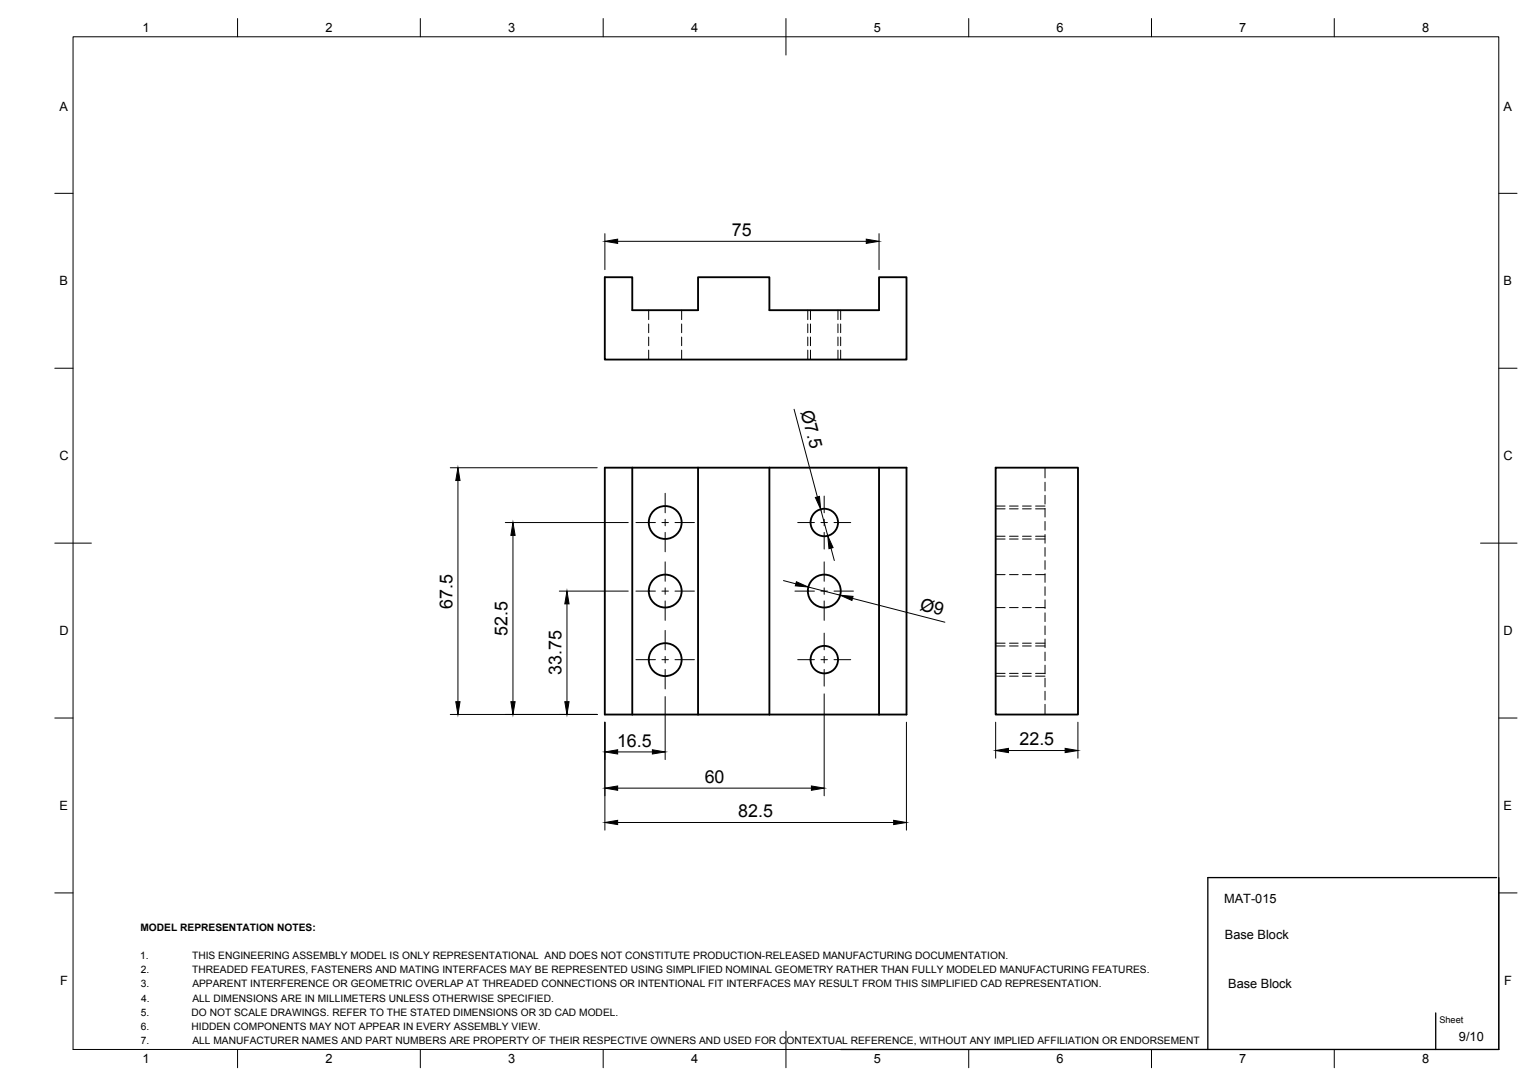
ISO-10303-21;
HEADER;
/* Generated by software containing ST-Developer
 * from STEP Tools, Inc. (www.steptools.com) 
 */

FILE_DESCRIPTION(
/* description */ ('STEP AP214'),
/* implementation_level */ '2;1');

FILE_NAME(
/* name */ 'Base Block.step',
/* time_stamp */ '2026-11-14T06:03:18-08:00',
/* author */ (''),
/* organization */ (''),
/* preprocessor_version */ 'ST-DEVELOPER v20.2',
/* originating_system */ 'Autodesk Translation Framework v15.17.0.0',
/* authorisation */ '');

FILE_SCHEMA (('AUTOMOTIVE_DESIGN { 1 0 10303 214 3 1 1 }'));
ENDSEC;

DATA;
#10=MECHANICAL_DESIGN_GEOMETRIC_PRESENTATION_REPRESENTATION('',(#77),#3206);
#61=SHAPE_REPRESENTATION_RELATIONSHIP('SRR','None',#3244,#69);
#69=ADVANCED_BREP_SHAPE_REPRESENTATION('',(#85),#3203);
#77=STYLED_ITEM('',(#3289),#85);
#85=MANIFOLD_SOLID_BREP('Body1',#1784);
#117=PLANE('',#2002);
#118=PLANE('',#2003);
#119=PLANE('',#2004);
#120=PLANE('',#2005);
#121=PLANE('',#2006);
#122=PLANE('',#2007);
#123=PLANE('',#2008);
#124=PLANE('',#2009);
#125=PLANE('',#2010);
#126=PLANE('',#2011);
#127=PLANE('',#2012);
#128=PLANE('',#2013);
#129=PLANE('',#2014);
#130=PLANE('',#2015);
#168=FACE_BOUND('',#693,.T.);
#169=FACE_BOUND('',#694,.T.);
#170=FACE_BOUND('',#695,.T.);
#171=FACE_BOUND('',#697,.T.);
#172=FACE_BOUND('',#698,.T.);
#173=FACE_BOUND('',#699,.T.);
#174=FACE_BOUND('',#701,.T.);
#175=FACE_BOUND('',#702,.T.);
#176=FACE_BOUND('',#703,.T.);
#177=FACE_BOUND('',#704,.T.);
#178=FACE_BOUND('',#705,.T.);
#179=FACE_BOUND('',#706,.T.);
#244=LINE('',#2930,#389);
#245=LINE('',#2936,#390);
#246=LINE('',#2942,#391);
#247=LINE('',#2948,#392);
#248=LINE('',#2954,#393);
#249=LINE('',#2960,#394);
#250=LINE('',#2965,#395);
#251=LINE('',#2967,#396);
#252=LINE('',#2969,#397);
#253=LINE('',#2970,#398);
#254=LINE('',#2974,#399);
#255=LINE('',#2976,#400);
#256=LINE('',#2978,#401);
#257=LINE('',#2979,#402);
#258=LINE('',#2983,#403);
#259=LINE('',#2985,#404);
#260=LINE('',#2987,#405);
#261=LINE('',#2988,#406);
#262=LINE('',#2991,#407);
#263=LINE('',#2993,#408);
#264=LINE('',#2994,#409);
#265=LINE('',#2997,#410);
#266=LINE('',#2999,#411);
#267=LINE('',#3000,#412);
#268=LINE('',#3002,#413);
#269=LINE('',#3004,#414);
#270=LINE('',#3005,#415);
#271=LINE('',#3007,#416);
#272=LINE('',#3008,#417);
#273=LINE('',#3011,#418);
#274=LINE('',#3012,#419);
#275=LINE('',#3015,#420);
#276=LINE('',#3016,#421);
#277=LINE('',#3018,#422);
#278=LINE('',#3020,#423);
#279=LINE('',#3021,#424);
#280=LINE('',#3023,#425);
#281=LINE('',#3024,#426);
#282=LINE('',#3026,#427);
#283=LINE('',#3028,#428);
#284=LINE('',#3031,#429);
#285=LINE('',#3034,#430);
#389=VECTOR('',#2351,4.5);
#390=VECTOR('',#2358,4.5);
#391=VECTOR('',#2365,4.5);
#392=VECTOR('',#2372,4.5);
#393=VECTOR('',#2379,3.75);
#394=VECTOR('',#2386,3.75);
#395=VECTOR('',#2391,1000.);
#396=VECTOR('',#2392,1000.);
#397=VECTOR('',#2393,1000.);
#398=VECTOR('',#2394,1000.);
#399=VECTOR('',#2397,1000.);
#400=VECTOR('',#2398,1000.);
#401=VECTOR('',#2399,1000.);
#402=VECTOR('',#2400,1000.);
#403=VECTOR('',#2403,1000.);
#404=VECTOR('',#2404,1000.);
#405=VECTOR('',#2405,1000.);
#406=VECTOR('',#2406,1000.);
#407=VECTOR('',#2409,1000.);
#408=VECTOR('',#2410,1000.);
#409=VECTOR('',#2411,1000.);
#410=VECTOR('',#2414,1000.);
#411=VECTOR('',#2415,1000.);
#412=VECTOR('',#2416,1000.);
#413=VECTOR('',#2417,1000.);
#414=VECTOR('',#2418,1000.);
#415=VECTOR('',#2419,1000.);
#416=VECTOR('',#2420,1000.);
#417=VECTOR('',#2421,1000.);
#418=VECTOR('',#2424,1000.);
#419=VECTOR('',#2425,1000.);
#420=VECTOR('',#2428,1000.);
#421=VECTOR('',#2429,1000.);
#422=VECTOR('',#2430,1000.);
#423=VECTOR('',#2431,1000.);
#424=VECTOR('',#2432,1000.);
#425=VECTOR('',#2433,1000.);
#426=VECTOR('',#2434,1000.);
#427=VECTOR('',#2437,1000.);
#428=VECTOR('',#2440,1000.);
#429=VECTOR('',#2445,1000.);
#430=VECTOR('',#2450,1000.);
#497=CYLINDRICAL_SURFACE('',#1984,4.5);
#498=CYLINDRICAL_SURFACE('',#1987,4.5);
#499=CYLINDRICAL_SURFACE('',#1990,4.5);
#500=CYLINDRICAL_SURFACE('',#1993,4.5);
#501=CYLINDRICAL_SURFACE('',#1996,3.75);
#502=CYLINDRICAL_SURFACE('',#1999,3.75);
#565=FACE_OUTER_BOUND('',#686,.T.);
#566=FACE_OUTER_BOUND('',#687,.T.);
#567=FACE_OUTER_BOUND('',#688,.T.);
#568=FACE_OUTER_BOUND('',#689,.T.);
#569=FACE_OUTER_BOUND('',#690,.T.);
#570=FACE_OUTER_BOUND('',#691,.T.);
#571=FACE_OUTER_BOUND('',#692,.T.);
#572=FACE_OUTER_BOUND('',#696,.T.);
#573=FACE_OUTER_BOUND('',#700,.T.);
#574=FACE_OUTER_BOUND('',#707,.T.);
#575=FACE_OUTER_BOUND('',#708,.T.);
#576=FACE_OUTER_BOUND('',#709,.T.);
#577=FACE_OUTER_BOUND('',#710,.T.);
#578=FACE_OUTER_BOUND('',#711,.T.);
#579=FACE_OUTER_BOUND('',#712,.T.);
#580=FACE_OUTER_BOUND('',#713,.T.);
#581=FACE_OUTER_BOUND('',#714,.T.);
#582=FACE_OUTER_BOUND('',#715,.T.);
#583=FACE_OUTER_BOUND('',#716,.T.);
#584=FACE_OUTER_BOUND('',#717,.T.);
#686=EDGE_LOOP('',(#1433,#1434,#1435,#1436));
#687=EDGE_LOOP('',(#1437,#1438,#1439,#1440));
#688=EDGE_LOOP('',(#1441,#1442,#1443,#1444));
#689=EDGE_LOOP('',(#1445,#1446,#1447,#1448));
#690=EDGE_LOOP('',(#1449,#1450,#1451,#1452));
#691=EDGE_LOOP('',(#1453,#1454,#1455,#1456));
#692=EDGE_LOOP('',(#1457,#1458,#1459,#1460));
#693=EDGE_LOOP('',(#1461));
#694=EDGE_LOOP('',(#1462));
#695=EDGE_LOOP('',(#1463));
#696=EDGE_LOOP('',(#1464,#1465,#1466,#1467));
#697=EDGE_LOOP('',(#1468));
#698=EDGE_LOOP('',(#1469));
#699=EDGE_LOOP('',(#1470));
#700=EDGE_LOOP('',(#1471,#1472,#1473,#1474));
#701=EDGE_LOOP('',(#1475));
#702=EDGE_LOOP('',(#1476));
#703=EDGE_LOOP('',(#1477));
#704=EDGE_LOOP('',(#1478));
#705=EDGE_LOOP('',(#1479));
#706=EDGE_LOOP('',(#1480));
#707=EDGE_LOOP('',(#1481,#1482,#1483,#1484));
#708=EDGE_LOOP('',(#1485,#1486,#1487,#1488,#1489,#1490,#1491,#1492,#1493,
#1494,#1495,#1496));
#709=EDGE_LOOP('',(#1497,#1498,#1499,#1500));
#710=EDGE_LOOP('',(#1501,#1502,#1503,#1504,#1505,#1506,#1507,#1508,#1509,
#1510,#1511,#1512));
#711=EDGE_LOOP('',(#1513,#1514,#1515,#1516));
#712=EDGE_LOOP('',(#1517,#1518,#1519,#1520));
#713=EDGE_LOOP('',(#1521,#1522,#1523,#1524));
#714=EDGE_LOOP('',(#1525,#1526,#1527,#1528));
#715=EDGE_LOOP('',(#1529,#1530,#1531,#1532));
#716=EDGE_LOOP('',(#1533,#1534,#1535,#1536));
#717=EDGE_LOOP('',(#1537,#1538,#1539,#1540));
#801=CIRCLE('',#1985,4.5);
#802=CIRCLE('',#1986,4.5);
#803=CIRCLE('',#1988,4.5);
#804=CIRCLE('',#1989,4.5);
#805=CIRCLE('',#1991,4.5);
#806=CIRCLE('',#1992,4.5);
#807=CIRCLE('',#1994,4.5);
#808=CIRCLE('',#1995,4.5);
#809=CIRCLE('',#1997,3.75);
#810=CIRCLE('',#1998,3.75);
#811=CIRCLE('',#2000,3.75);
#812=CIRCLE('',#2001,3.75);
#906=VERTEX_POINT('',#2927);
#907=VERTEX_POINT('',#2929);
#908=VERTEX_POINT('',#2933);
#909=VERTEX_POINT('',#2935);
#910=VERTEX_POINT('',#2939);
#911=VERTEX_POINT('',#2941);
#912=VERTEX_POINT('',#2945);
#913=VERTEX_POINT('',#2947);
#914=VERTEX_POINT('',#2951);
#915=VERTEX_POINT('',#2953);
#916=VERTEX_POINT('',#2957);
#917=VERTEX_POINT('',#2959);
#918=VERTEX_POINT('',#2963);
#919=VERTEX_POINT('',#2964);
#920=VERTEX_POINT('',#2966);
#921=VERTEX_POINT('',#2968);
#922=VERTEX_POINT('',#2972);
#923=VERTEX_POINT('',#2973);
#924=VERTEX_POINT('',#2975);
#925=VERTEX_POINT('',#2977);
#926=VERTEX_POINT('',#2981);
#927=VERTEX_POINT('',#2982);
#928=VERTEX_POINT('',#2984);
#929=VERTEX_POINT('',#2986);
#930=VERTEX_POINT('',#2990);
#931=VERTEX_POINT('',#2992);
#932=VERTEX_POINT('',#2996);
#933=VERTEX_POINT('',#2998);
#934=VERTEX_POINT('',#3001);
#935=VERTEX_POINT('',#3003);
#936=VERTEX_POINT('',#3006);
#937=VERTEX_POINT('',#3010);
#938=VERTEX_POINT('',#3014);
#939=VERTEX_POINT('',#3017);
#940=VERTEX_POINT('',#3019);
#941=VERTEX_POINT('',#3022);
#1095=EDGE_CURVE('',#906,#906,#801,.T.);
#1096=EDGE_CURVE('',#906,#907,#244,.T.);
#1097=EDGE_CURVE('',#907,#907,#802,.T.);
#1098=EDGE_CURVE('',#908,#908,#803,.T.);
#1099=EDGE_CURVE('',#908,#909,#245,.T.);
#1100=EDGE_CURVE('',#909,#909,#804,.T.);
#1101=EDGE_CURVE('',#910,#910,#805,.T.);
#1102=EDGE_CURVE('',#910,#911,#246,.T.);
#1103=EDGE_CURVE('',#911,#911,#806,.T.);
#1104=EDGE_CURVE('',#912,#912,#807,.T.);
#1105=EDGE_CURVE('',#912,#913,#247,.T.);
#1106=EDGE_CURVE('',#913,#913,#808,.T.);
#1107=EDGE_CURVE('',#914,#914,#809,.T.);
#1108=EDGE_CURVE('',#914,#915,#248,.T.);
#1109=EDGE_CURVE('',#915,#915,#810,.T.);
#1110=EDGE_CURVE('',#916,#916,#811,.T.);
#1111=EDGE_CURVE('',#916,#917,#249,.T.);
#1112=EDGE_CURVE('',#917,#917,#812,.T.);
#1113=EDGE_CURVE('',#918,#919,#250,.T.);
#1114=EDGE_CURVE('',#919,#920,#251,.T.);
#1115=EDGE_CURVE('',#920,#921,#252,.T.);
#1116=EDGE_CURVE('',#921,#918,#253,.T.);
#1117=EDGE_CURVE('',#922,#923,#254,.T.);
#1118=EDGE_CURVE('',#923,#924,#255,.T.);
#1119=EDGE_CURVE('',#924,#925,#256,.T.);
#1120=EDGE_CURVE('',#925,#922,#257,.T.);
#1121=EDGE_CURVE('',#926,#927,#258,.T.);
#1122=EDGE_CURVE('',#928,#926,#259,.T.);
#1123=EDGE_CURVE('',#929,#928,#260,.T.);
#1124=EDGE_CURVE('',#927,#929,#261,.T.);
#1125=EDGE_CURVE('',#930,#927,#262,.T.);
#1126=EDGE_CURVE('',#931,#930,#263,.T.);
#1127=EDGE_CURVE('',#931,#926,#264,.T.);
#1128=EDGE_CURVE('',#932,#929,#265,.T.);
#1129=EDGE_CURVE('',#933,#932,#266,.T.);
#1130=EDGE_CURVE('',#933,#918,#267,.T.);
#1131=EDGE_CURVE('',#934,#921,#268,.T.);
#1132=EDGE_CURVE('',#935,#934,#269,.T.);
#1133=EDGE_CURVE('',#935,#924,#270,.T.);
#1134=EDGE_CURVE('',#936,#923,#271,.T.);
#1135=EDGE_CURVE('',#930,#936,#272,.T.);
#1136=EDGE_CURVE('',#937,#928,#273,.T.);
#1137=EDGE_CURVE('',#932,#937,#274,.T.);
#1138=EDGE_CURVE('',#938,#931,#275,.T.);
#1139=EDGE_CURVE('',#938,#922,#276,.T.);
#1140=EDGE_CURVE('',#939,#925,#277,.T.);
#1141=EDGE_CURVE('',#940,#939,#278,.T.);
#1142=EDGE_CURVE('',#940,#920,#279,.T.);
#1143=EDGE_CURVE('',#941,#919,#280,.T.);
#1144=EDGE_CURVE('',#937,#941,#281,.T.);
#1145=EDGE_CURVE('',#940,#934,#282,.T.);
#1146=EDGE_CURVE('',#935,#939,#283,.T.);
#1147=EDGE_CURVE('',#933,#941,#284,.T.);
#1148=EDGE_CURVE('',#938,#936,#285,.T.);
#1433=ORIENTED_EDGE('',*,*,#1095,.T.);
#1434=ORIENTED_EDGE('',*,*,#1096,.T.);
#1435=ORIENTED_EDGE('',*,*,#1097,.F.);
#1436=ORIENTED_EDGE('',*,*,#1096,.F.);
#1437=ORIENTED_EDGE('',*,*,#1098,.T.);
#1438=ORIENTED_EDGE('',*,*,#1099,.T.);
#1439=ORIENTED_EDGE('',*,*,#1100,.F.);
#1440=ORIENTED_EDGE('',*,*,#1099,.F.);
#1441=ORIENTED_EDGE('',*,*,#1101,.T.);
#1442=ORIENTED_EDGE('',*,*,#1102,.T.);
#1443=ORIENTED_EDGE('',*,*,#1103,.F.);
#1444=ORIENTED_EDGE('',*,*,#1102,.F.);
#1445=ORIENTED_EDGE('',*,*,#1104,.T.);
#1446=ORIENTED_EDGE('',*,*,#1105,.T.);
#1447=ORIENTED_EDGE('',*,*,#1106,.F.);
#1448=ORIENTED_EDGE('',*,*,#1105,.F.);
#1449=ORIENTED_EDGE('',*,*,#1107,.T.);
#1450=ORIENTED_EDGE('',*,*,#1108,.T.);
#1451=ORIENTED_EDGE('',*,*,#1109,.F.);
#1452=ORIENTED_EDGE('',*,*,#1108,.F.);
#1453=ORIENTED_EDGE('',*,*,#1110,.T.);
#1454=ORIENTED_EDGE('',*,*,#1111,.T.);
#1455=ORIENTED_EDGE('',*,*,#1112,.F.);
#1456=ORIENTED_EDGE('',*,*,#1111,.F.);
#1457=ORIENTED_EDGE('',*,*,#1113,.T.);
#1458=ORIENTED_EDGE('',*,*,#1114,.T.);
#1459=ORIENTED_EDGE('',*,*,#1115,.T.);
#1460=ORIENTED_EDGE('',*,*,#1116,.T.);
#1461=ORIENTED_EDGE('',*,*,#1107,.F.);
#1462=ORIENTED_EDGE('',*,*,#1110,.F.);
#1463=ORIENTED_EDGE('',*,*,#1104,.F.);
#1464=ORIENTED_EDGE('',*,*,#1117,.T.);
#1465=ORIENTED_EDGE('',*,*,#1118,.T.);
#1466=ORIENTED_EDGE('',*,*,#1119,.T.);
#1467=ORIENTED_EDGE('',*,*,#1120,.T.);
#1468=ORIENTED_EDGE('',*,*,#1095,.F.);
#1469=ORIENTED_EDGE('',*,*,#1101,.F.);
#1470=ORIENTED_EDGE('',*,*,#1098,.F.);
#1471=ORIENTED_EDGE('',*,*,#1121,.F.);
#1472=ORIENTED_EDGE('',*,*,#1122,.F.);
#1473=ORIENTED_EDGE('',*,*,#1123,.F.);
#1474=ORIENTED_EDGE('',*,*,#1124,.F.);
#1475=ORIENTED_EDGE('',*,*,#1109,.T.);
#1476=ORIENTED_EDGE('',*,*,#1103,.T.);
#1477=ORIENTED_EDGE('',*,*,#1097,.T.);
#1478=ORIENTED_EDGE('',*,*,#1100,.T.);
#1479=ORIENTED_EDGE('',*,*,#1106,.T.);
#1480=ORIENTED_EDGE('',*,*,#1112,.T.);
#1481=ORIENTED_EDGE('',*,*,#1121,.T.);
#1482=ORIENTED_EDGE('',*,*,#1125,.F.);
#1483=ORIENTED_EDGE('',*,*,#1126,.F.);
#1484=ORIENTED_EDGE('',*,*,#1127,.T.);
#1485=ORIENTED_EDGE('',*,*,#1124,.T.);
#1486=ORIENTED_EDGE('',*,*,#1128,.F.);
#1487=ORIENTED_EDGE('',*,*,#1129,.F.);
#1488=ORIENTED_EDGE('',*,*,#1130,.T.);
#1489=ORIENTED_EDGE('',*,*,#1116,.F.);
#1490=ORIENTED_EDGE('',*,*,#1131,.F.);
#1491=ORIENTED_EDGE('',*,*,#1132,.F.);
#1492=ORIENTED_EDGE('',*,*,#1133,.T.);
#1493=ORIENTED_EDGE('',*,*,#1118,.F.);
#1494=ORIENTED_EDGE('',*,*,#1134,.F.);
#1495=ORIENTED_EDGE('',*,*,#1135,.F.);
#1496=ORIENTED_EDGE('',*,*,#1125,.T.);
#1497=ORIENTED_EDGE('',*,*,#1123,.T.);
#1498=ORIENTED_EDGE('',*,*,#1136,.F.);
#1499=ORIENTED_EDGE('',*,*,#1137,.F.);
#1500=ORIENTED_EDGE('',*,*,#1128,.T.);
#1501=ORIENTED_EDGE('',*,*,#1122,.T.);
#1502=ORIENTED_EDGE('',*,*,#1127,.F.);
#1503=ORIENTED_EDGE('',*,*,#1138,.F.);
#1504=ORIENTED_EDGE('',*,*,#1139,.T.);
#1505=ORIENTED_EDGE('',*,*,#1120,.F.);
#1506=ORIENTED_EDGE('',*,*,#1140,.F.);
#1507=ORIENTED_EDGE('',*,*,#1141,.F.);
#1508=ORIENTED_EDGE('',*,*,#1142,.T.);
#1509=ORIENTED_EDGE('',*,*,#1114,.F.);
#1510=ORIENTED_EDGE('',*,*,#1143,.F.);
#1511=ORIENTED_EDGE('',*,*,#1144,.F.);
#1512=ORIENTED_EDGE('',*,*,#1136,.T.);
#1513=ORIENTED_EDGE('',*,*,#1115,.F.);
#1514=ORIENTED_EDGE('',*,*,#1142,.F.);
#1515=ORIENTED_EDGE('',*,*,#1145,.T.);
#1516=ORIENTED_EDGE('',*,*,#1131,.T.);
#1517=ORIENTED_EDGE('',*,*,#1119,.F.);
#1518=ORIENTED_EDGE('',*,*,#1133,.F.);
#1519=ORIENTED_EDGE('',*,*,#1146,.T.);
#1520=ORIENTED_EDGE('',*,*,#1140,.T.);
#1521=ORIENTED_EDGE('',*,*,#1145,.F.);
#1522=ORIENTED_EDGE('',*,*,#1141,.T.);
#1523=ORIENTED_EDGE('',*,*,#1146,.F.);
#1524=ORIENTED_EDGE('',*,*,#1132,.T.);
#1525=ORIENTED_EDGE('',*,*,#1113,.F.);
#1526=ORIENTED_EDGE('',*,*,#1130,.F.);
#1527=ORIENTED_EDGE('',*,*,#1147,.T.);
#1528=ORIENTED_EDGE('',*,*,#1143,.T.);
#1529=ORIENTED_EDGE('',*,*,#1147,.F.);
#1530=ORIENTED_EDGE('',*,*,#1129,.T.);
#1531=ORIENTED_EDGE('',*,*,#1137,.T.);
#1532=ORIENTED_EDGE('',*,*,#1144,.T.);
#1533=ORIENTED_EDGE('',*,*,#1117,.F.);
#1534=ORIENTED_EDGE('',*,*,#1139,.F.);
#1535=ORIENTED_EDGE('',*,*,#1148,.T.);
#1536=ORIENTED_EDGE('',*,*,#1134,.T.);
#1537=ORIENTED_EDGE('',*,*,#1148,.F.);
#1538=ORIENTED_EDGE('',*,*,#1138,.T.);
#1539=ORIENTED_EDGE('',*,*,#1126,.T.);
#1540=ORIENTED_EDGE('',*,*,#1135,.T.);
#1732=ADVANCED_FACE('',(#565),#497,.F.);
#1733=ADVANCED_FACE('',(#566),#498,.F.);
#1734=ADVANCED_FACE('',(#567),#499,.F.);
#1735=ADVANCED_FACE('',(#568),#500,.F.);
#1736=ADVANCED_FACE('',(#569),#501,.F.);
#1737=ADVANCED_FACE('',(#570),#502,.F.);
#1738=ADVANCED_FACE('',(#571,#168,#169,#170),#117,.T.);
#1739=ADVANCED_FACE('',(#572,#171,#172,#173),#118,.T.);
#1740=ADVANCED_FACE('',(#573,#174,#175,#176,#177,#178,#179),#119,.F.);
#1741=ADVANCED_FACE('',(#574),#120,.F.);
#1742=ADVANCED_FACE('',(#575),#121,.F.);
#1743=ADVANCED_FACE('',(#576),#122,.F.);
#1744=ADVANCED_FACE('',(#577),#123,.F.);
#1745=ADVANCED_FACE('',(#578),#124,.T.);
#1746=ADVANCED_FACE('',(#579),#125,.T.);
#1747=ADVANCED_FACE('',(#580),#126,.T.);
#1748=ADVANCED_FACE('',(#581),#127,.T.);
#1749=ADVANCED_FACE('',(#582),#128,.T.);
#1750=ADVANCED_FACE('',(#583),#129,.T.);
#1751=ADVANCED_FACE('',(#584),#130,.T.);
#1784=CLOSED_SHELL('',(#1732,#1733,#1734,#1735,#1736,#1737,#1738,#1739,
#1740,#1741,#1742,#1743,#1744,#1745,#1746,#1747,#1748,#1749,#1750,#1751));
#1983=AXIS2_PLACEMENT_3D('',#2925,#2345,#2346);
#1984=AXIS2_PLACEMENT_3D('',#2926,#2347,#2348);
#1985=AXIS2_PLACEMENT_3D('',#2928,#2349,#2350);
#1986=AXIS2_PLACEMENT_3D('',#2931,#2352,#2353);
#1987=AXIS2_PLACEMENT_3D('',#2932,#2354,#2355);
#1988=AXIS2_PLACEMENT_3D('',#2934,#2356,#2357);
#1989=AXIS2_PLACEMENT_3D('',#2937,#2359,#2360);
#1990=AXIS2_PLACEMENT_3D('',#2938,#2361,#2362);
#1991=AXIS2_PLACEMENT_3D('',#2940,#2363,#2364);
#1992=AXIS2_PLACEMENT_3D('',#2943,#2366,#2367);
#1993=AXIS2_PLACEMENT_3D('',#2944,#2368,#2369);
#1994=AXIS2_PLACEMENT_3D('',#2946,#2370,#2371);
#1995=AXIS2_PLACEMENT_3D('',#2949,#2373,#2374);
#1996=AXIS2_PLACEMENT_3D('',#2950,#2375,#2376);
#1997=AXIS2_PLACEMENT_3D('',#2952,#2377,#2378);
#1998=AXIS2_PLACEMENT_3D('',#2955,#2380,#2381);
#1999=AXIS2_PLACEMENT_3D('',#2956,#2382,#2383);
#2000=AXIS2_PLACEMENT_3D('',#2958,#2384,#2385);
#2001=AXIS2_PLACEMENT_3D('',#2961,#2387,#2388);
#2002=AXIS2_PLACEMENT_3D('',#2962,#2389,#2390);
#2003=AXIS2_PLACEMENT_3D('',#2971,#2395,#2396);
#2004=AXIS2_PLACEMENT_3D('',#2980,#2401,#2402);
#2005=AXIS2_PLACEMENT_3D('',#2989,#2407,#2408);
#2006=AXIS2_PLACEMENT_3D('',#2995,#2412,#2413);
#2007=AXIS2_PLACEMENT_3D('',#3009,#2422,#2423);
#2008=AXIS2_PLACEMENT_3D('',#3013,#2426,#2427);
#2009=AXIS2_PLACEMENT_3D('',#3025,#2435,#2436);
#2010=AXIS2_PLACEMENT_3D('',#3027,#2438,#2439);
#2011=AXIS2_PLACEMENT_3D('',#3029,#2441,#2442);
#2012=AXIS2_PLACEMENT_3D('',#3030,#2443,#2444);
#2013=AXIS2_PLACEMENT_3D('',#3032,#2446,#2447);
#2014=AXIS2_PLACEMENT_3D('',#3033,#2448,#2449);
#2015=AXIS2_PLACEMENT_3D('',#3035,#2451,#2452);
#2345=DIRECTION('axis',(0.,0.,1.));
#2346=DIRECTION('refdir',(1.,0.,0.));
#2347=DIRECTION('center_axis',(1.46707713513697E-31,-1.04083408558608E-17,
-1.));
#2348=DIRECTION('ref_axis',(-1.,-1.52698388843454E-48,-1.46707713513697E-31));
#2349=DIRECTION('center_axis',(-1.46707713513697E-31,1.04083408558608E-17,
1.));
#2350=DIRECTION('ref_axis',(-1.,-1.52698388843454E-48,-1.46707713513697E-31));
#2351=DIRECTION('',(1.46707713513697E-31,-1.04083408558608E-17,-1.));
#2352=DIRECTION('center_axis',(-1.46707713513697E-31,1.04083408558608E-17,
1.));
#2353=DIRECTION('ref_axis',(-1.,-1.52698388843454E-48,-1.46707713513697E-31));
#2354=DIRECTION('center_axis',(1.46707713513697E-31,-1.04083408558608E-17,
-1.));
#2355=DIRECTION('ref_axis',(-1.,-1.52698388843454E-48,-1.46707713513697E-31));
#2356=DIRECTION('center_axis',(-1.46707713513697E-31,1.04083408558608E-17,
1.));
#2357=DIRECTION('ref_axis',(-1.,-1.52698388843454E-48,-1.46707713513697E-31));
#2358=DIRECTION('',(1.46707713513697E-31,-1.04083408558608E-17,-1.));
#2359=DIRECTION('center_axis',(-1.46707713513697E-31,1.04083408558608E-17,
1.));
#2360=DIRECTION('ref_axis',(-1.,-1.52698388843454E-48,-1.46707713513697E-31));
#2361=DIRECTION('center_axis',(1.46707713513697E-31,-1.04083408558608E-17,
-1.));
#2362=DIRECTION('ref_axis',(-1.,-1.52698388843454E-48,-1.46707713513697E-31));
#2363=DIRECTION('center_axis',(-1.46707713513697E-31,1.04083408558608E-17,
1.));
#2364=DIRECTION('ref_axis',(-1.,-1.52698388843454E-48,-1.46707713513697E-31));
#2365=DIRECTION('',(1.46707713513697E-31,-1.04083408558608E-17,-1.));
#2366=DIRECTION('center_axis',(-1.46707713513697E-31,1.04083408558608E-17,
1.));
#2367=DIRECTION('ref_axis',(-1.,-1.52698388843454E-48,-1.46707713513697E-31));
#2368=DIRECTION('center_axis',(1.46707713513697E-31,-1.04083408558608E-17,
-1.));
#2369=DIRECTION('ref_axis',(-1.,-1.52698388843454E-48,-1.46707713513697E-31));
#2370=DIRECTION('center_axis',(-1.46707713513697E-31,1.04083408558608E-17,
1.));
#2371=DIRECTION('ref_axis',(1.,1.52698388843454E-48,1.46707713513697E-31));
#2372=DIRECTION('',(1.46707713513697E-31,-1.04083408558608E-17,-1.));
#2373=DIRECTION('center_axis',(-1.46707713513697E-31,1.04083408558608E-17,
1.));
#2374=DIRECTION('ref_axis',(1.,1.52698388843454E-48,1.46707713513697E-31));
#2375=DIRECTION('center_axis',(1.46707713513697E-31,-1.04083408558608E-17,
-1.));
#2376=DIRECTION('ref_axis',(-1.,-1.52698388843454E-48,-1.46707713513697E-31));
#2377=DIRECTION('center_axis',(-1.46707713513697E-31,1.04083408558608E-17,
1.));
#2378=DIRECTION('ref_axis',(1.,1.52698388843454E-48,1.46707713513697E-31));
#2379=DIRECTION('',(1.46707713513697E-31,-1.04083408558608E-17,-1.));
#2380=DIRECTION('center_axis',(-1.46707713513697E-31,1.04083408558608E-17,
1.));
#2381=DIRECTION('ref_axis',(1.,1.52698388843454E-48,1.46707713513697E-31));
#2382=DIRECTION('center_axis',(1.46707713513697E-31,-1.04083408558608E-17,
-1.));
#2383=DIRECTION('ref_axis',(-1.,-1.52698388843454E-48,-1.46707713513697E-31));
#2384=DIRECTION('center_axis',(-1.46707713513697E-31,1.04083408558608E-17,
1.));
#2385=DIRECTION('ref_axis',(1.,1.52698388843454E-48,1.46707713513697E-31));
#2386=DIRECTION('',(1.46707713513697E-31,-1.04083408558608E-17,-1.));
#2387=DIRECTION('center_axis',(-1.46707713513697E-31,1.04083408558608E-17,
1.));
#2388=DIRECTION('ref_axis',(1.,1.52698388843454E-48,1.46707713513697E-31));
#2389=DIRECTION('center_axis',(1.46659565265088E-31,1.04083408558608E-17,
1.));
#2390=DIRECTION('ref_axis',(1.,-2.77333911991762E-32,-1.46659565265088E-31));
#2391=DIRECTION('',(1.15648231731787E-16,-1.,1.04083408558608E-17));
#2392=DIRECTION('',(1.,-2.77333911991762E-32,-1.46659565265088E-31));
#2393=DIRECTION('',(-2.92741351546859E-32,1.,-1.04083408558608E-17));
#2394=DIRECTION('',(-1.,2.77333911991762E-32,1.46659565265088E-31));
#2395=DIRECTION('center_axis',(1.46659565265088E-31,1.04083408558608E-17,
1.));
#2396=DIRECTION('ref_axis',(1.,-2.77333911991762E-32,-1.46659565265088E-31));
#2397=DIRECTION('',(-2.92741351546859E-32,1.,-1.04083408558608E-17));
#2398=DIRECTION('',(-1.,2.77333911991762E-32,1.46659565265088E-31));
#2399=DIRECTION('',(2.92741351546859E-32,-1.,1.04083408558608E-17));
#2400=DIRECTION('',(1.,-2.77333911991762E-32,-1.46659565265088E-31));
#2401=DIRECTION('center_axis',(1.46659565265088E-31,1.04083408558608E-17,
1.));
#2402=DIRECTION('ref_axis',(1.,-2.77333911991762E-32,-1.46659565265088E-31));
#2403=DIRECTION('',(-2.92741351546859E-32,1.,-6.93889390390721E-18));
#2404=DIRECTION('',(1.,-2.77333911991762E-32,-1.46659565265088E-31));
#2405=DIRECTION('',(2.92741351546859E-32,-1.,6.93889390390721E-18));
#2406=DIRECTION('',(-1.,2.77333911991762E-32,1.46659565265088E-31));
#2407=DIRECTION('center_axis',(-1.,2.77333911991762E-32,-1.46707713513697E-31));
#2408=DIRECTION('ref_axis',(-1.46707713513697E-31,1.04083408558608E-17,
1.));
#2409=DIRECTION('',(1.46707713513697E-31,-1.04083408558608E-17,-1.));
#2410=DIRECTION('',(-2.92741351546859E-32,1.,-1.04083408558608E-17));
#2411=DIRECTION('',(1.46707713513697E-31,-1.04083408558608E-17,-1.));
#2412=DIRECTION('center_axis',(2.92741351546859E-32,-1.,1.04083408558608E-17));
#2413=DIRECTION('ref_axis',(1.46707713513697E-31,-1.04083408558608E-17,
-1.));
#2414=DIRECTION('',(1.46707713513697E-31,-1.04083408558608E-17,-1.));
#2415=DIRECTION('',(-1.,2.77333911991762E-32,1.46659565265088E-31));
#2416=DIRECTION('',(1.46707713513697E-31,-1.04083408558608E-17,-1.));
#2417=DIRECTION('',(1.46707713513697E-31,-1.04083408558608E-17,-1.));
#2418=DIRECTION('',(-1.,2.77333911991762E-32,1.46659565265088E-31));
#2419=DIRECTION('',(1.46707713513697E-31,-1.04083408558608E-17,-1.));
#2420=DIRECTION('',(1.46707713513697E-31,-1.04083408558608E-17,-1.));
#2421=DIRECTION('',(-1.,2.77333911991762E-32,1.46659565265088E-31));
#2422=DIRECTION('center_axis',(1.,-2.77333911991762E-32,1.46707713513697E-31));
#2423=DIRECTION('ref_axis',(1.46707713513697E-31,-1.04083408558608E-17,
-1.));
#2424=DIRECTION('',(1.46707713513697E-31,-1.04083408558608E-17,-1.));
#2425=DIRECTION('',(2.92741351546859E-32,-1.,1.04083408558608E-17));
#2426=DIRECTION('center_axis',(-2.92741351546859E-32,1.,-1.04083408558608E-17));
#2427=DIRECTION('ref_axis',(-1.46707713513697E-31,1.04083408558608E-17,
1.));
#2428=DIRECTION('',(1.,-2.77333911991762E-32,-1.46659565265088E-31));
#2429=DIRECTION('',(1.46707713513697E-31,-1.04083408558608E-17,-1.));
#2430=DIRECTION('',(1.46707713513697E-31,-1.04083408558608E-17,-1.));
#2431=DIRECTION('',(1.,-2.77333911991762E-32,-1.46659565265088E-31));
#2432=DIRECTION('',(1.46707713513697E-31,-1.04083408558608E-17,-1.));
#2433=DIRECTION('',(1.46707713513697E-31,-1.04083408558608E-17,-1.));
#2434=DIRECTION('',(1.,-2.77333911991762E-32,-1.46659565265088E-31));
#2435=DIRECTION('center_axis',(-1.,2.77333911991762E-32,-1.46707713513697E-31));
#2436=DIRECTION('ref_axis',(-1.46707713513697E-31,1.04083408558608E-17,
1.));
#2437=DIRECTION('',(-2.92741351546859E-32,1.,-1.04083408558608E-17));
#2438=DIRECTION('center_axis',(1.,-2.77333911991762E-32,1.46707713513697E-31));
#2439=DIRECTION('ref_axis',(1.46707713513697E-31,-1.04083408558608E-17,
-1.));
#2440=DIRECTION('',(2.92741351546859E-32,-1.,1.04083408558608E-17));
#2441=DIRECTION('center_axis',(1.46659565265088E-31,1.04083408558608E-17,
1.));
#2442=DIRECTION('ref_axis',(1.,-2.77333911991762E-32,-1.46659565265088E-31));
#2443=DIRECTION('center_axis',(1.,1.15648231731787E-16,-1.22103958474151E-31));
#2444=DIRECTION('ref_axis',(-1.15648231731787E-16,1.,-1.04083408558608E-17));
#2445=DIRECTION('',(1.15648231731787E-16,-1.,1.04083408558608E-17));
#2446=DIRECTION('center_axis',(1.46659565265088E-31,1.04083408558608E-17,
1.));
#2447=DIRECTION('ref_axis',(1.,-2.77333911991762E-32,-1.46659565265088E-31));
#2448=DIRECTION('center_axis',(-1.,2.77333911991762E-32,-1.46707713513697E-31));
#2449=DIRECTION('ref_axis',(-1.46707713513697E-31,1.04083408558608E-17,
1.));
#2450=DIRECTION('',(-2.92741351546859E-32,1.,-1.04083408558608E-17));
#2451=DIRECTION('center_axis',(1.46659565265088E-31,1.04083408558608E-17,
1.));
#2452=DIRECTION('ref_axis',(1.,-2.77333911991762E-32,-1.46659565265088E-31));
#2925=CARTESIAN_POINT('',(0.,0.,0.));
#2926=CARTESIAN_POINT('Origin',(52.0832482616116,41.2500000000001,10.3911166878577));
#2927=CARTESIAN_POINT('',(56.5832482616116,41.2500000000001,10.3911166878577));
#2928=CARTESIAN_POINT('Origin',(52.0832482616116,41.2500000000001,10.3911166878577));
#2929=CARTESIAN_POINT('',(56.5832482616116,41.2500000000001,-3.10888331214233));
#2930=CARTESIAN_POINT('',(56.5832482616116,41.2500000000001,10.3911166878577));
#2931=CARTESIAN_POINT('Origin',(52.0832482616116,41.2500000000001,-3.10888331214233));
#2932=CARTESIAN_POINT('Origin',(52.0832482616116,3.75000000000002,10.3911166878578));
#2933=CARTESIAN_POINT('',(56.5832482616116,3.75000000000002,10.3911166878578));
#2934=CARTESIAN_POINT('Origin',(52.0832482616116,3.75000000000002,10.3911166878578));
#2935=CARTESIAN_POINT('',(56.5832482616116,3.75000000000002,-3.10888331214225));
#2936=CARTESIAN_POINT('',(56.5832482616116,3.75000000000002,10.3911166878578));
#2937=CARTESIAN_POINT('Origin',(52.0832482616116,3.75,-3.10888331214225));
#2938=CARTESIAN_POINT('Origin',(52.0832482616116,22.5,10.3911166878578));
#2939=CARTESIAN_POINT('',(56.5832482616116,22.5,10.3911166878578));
#2940=CARTESIAN_POINT('Origin',(52.0832482616116,22.5,10.3911166878578));
#2941=CARTESIAN_POINT('',(56.5832482616116,22.5,-3.10888331214233));
#2942=CARTESIAN_POINT('',(56.5832482616116,22.5,10.3911166878578));
#2943=CARTESIAN_POINT('Origin',(52.0832482616116,22.5,-3.10888331214233));
#2944=CARTESIAN_POINT('Origin',(8.5832482616116,22.5,10.3911166878578));
#2945=CARTESIAN_POINT('',(13.0832482616116,22.5,10.3911166878578));
#2946=CARTESIAN_POINT('Origin',(8.5832482616116,22.5,10.3911166878578));
#2947=CARTESIAN_POINT('',(13.0832482616116,22.5,-3.10888331214233));
#2948=CARTESIAN_POINT('',(13.0832482616116,22.5,10.3911166878578));
#2949=CARTESIAN_POINT('Origin',(8.5832482616116,22.5,-3.10888331214233));
#2950=CARTESIAN_POINT('Origin',(8.58324826161155,3.75000000000002,10.3911166878578));
#2951=CARTESIAN_POINT('',(12.3332482616116,3.75000000000002,10.3911166878578));
#2952=CARTESIAN_POINT('Origin',(8.58324826161155,3.75000000000002,10.3911166878578));
#2953=CARTESIAN_POINT('',(12.3332482616116,3.75000000000002,-3.10888331214225));
#2954=CARTESIAN_POINT('',(12.3332482616116,3.75000000000002,10.3911166878578));
#2955=CARTESIAN_POINT('Origin',(8.5832482616116,3.75,-3.10888331214225));
#2956=CARTESIAN_POINT('Origin',(8.5832482616116,41.2500000000001,10.3911166878578));
#2957=CARTESIAN_POINT('',(12.3332482616116,41.2500000000001,10.3911166878578));
#2958=CARTESIAN_POINT('Origin',(8.5832482616116,41.2500000000001,10.3911166878578));
#2959=CARTESIAN_POINT('',(12.3332482616116,41.2500000000001,-3.10888331214233));
#2960=CARTESIAN_POINT('',(12.3332482616116,41.2500000000001,10.3911166878578));
#2961=CARTESIAN_POINT('Origin',(8.5832482616116,41.2500000000001,-3.10888331214233));
#2962=CARTESIAN_POINT('Origin',(-13.9167517383884,-11.25,10.3911166878578));
#2963=CARTESIAN_POINT('',(-6.41675173838841,56.25,10.3911166878578));
#2964=CARTESIAN_POINT('',(-6.41675173838841,-11.25,10.3911166878578));
#2965=CARTESIAN_POINT('',(-6.41675173838841,-11.25,10.3911166878578));
#2966=CARTESIAN_POINT('',(23.5832482616121,-11.25,10.3911166878578));
#2967=CARTESIAN_POINT('',(-13.9167517383884,-11.25,10.3911166878578));
#2968=CARTESIAN_POINT('',(23.5832482616121,56.25,10.3911166878578));
#2969=CARTESIAN_POINT('',(23.5832482616121,-11.25,10.3911166878578));
#2970=CARTESIAN_POINT('',(68.5832482616116,56.25,10.3911166878577));
#2971=CARTESIAN_POINT('Origin',(-13.9167517383884,-11.25,10.3911166878578));
#2972=CARTESIAN_POINT('',(61.0832482616116,-11.25,10.3911166878578));
#2973=CARTESIAN_POINT('',(61.0832482616116,56.25,10.3911166878577));
#2974=CARTESIAN_POINT('',(61.0832482616116,-11.25,10.3911166878578));
#2975=CARTESIAN_POINT('',(43.0832482616116,56.25,10.3911166878577));
#2976=CARTESIAN_POINT('',(68.5832482616116,56.25,10.3911166878577));
#2977=CARTESIAN_POINT('',(43.0832482616116,-11.25,10.3911166878578));
#2978=CARTESIAN_POINT('',(43.0832482616116,-11.25,10.3911166878578));
#2979=CARTESIAN_POINT('',(-13.9167517383884,-11.25,10.3911166878578));
#2980=CARTESIAN_POINT('Origin',(-13.9167517383884,-11.25,-3.10888331214225));
#2981=CARTESIAN_POINT('',(68.5832482616116,-11.25,-3.10888331214226));
#2982=CARTESIAN_POINT('',(68.5832482616116,56.2500000000001,-3.10888331214233));
#2983=CARTESIAN_POINT('',(68.5832482616116,-11.25,-3.10888331214226));
#2984=CARTESIAN_POINT('',(-13.9167517383884,-11.25,-3.10888331214225));
#2985=CARTESIAN_POINT('',(-13.9167517383884,-11.25,-3.10888331214225));
#2986=CARTESIAN_POINT('',(-13.9167517383884,56.2500000000001,-3.10888331214232));
#2987=CARTESIAN_POINT('',(-13.9167517383884,56.2500000000001,-3.10888331214232));
#2988=CARTESIAN_POINT('',(68.5832482616116,56.2500000000001,-3.10888331214233));
#2989=CARTESIAN_POINT('Origin',(68.5832482616116,-11.25,10.3911166878578));
#2990=CARTESIAN_POINT('',(68.5832482616116,56.2500000000001,19.3911166878577));
#2991=CARTESIAN_POINT('',(68.5832482616116,56.25,10.3911166878577));
#2992=CARTESIAN_POINT('',(68.5832482616116,-11.25,19.3911166878577));
#2993=CARTESIAN_POINT('',(68.5832482616116,-11.25,19.3911166878577));
#2994=CARTESIAN_POINT('',(68.5832482616116,-11.25,10.3911166878578));
#2995=CARTESIAN_POINT('Origin',(68.5832482616116,56.25,10.3911166878577));
#2996=CARTESIAN_POINT('',(-13.9167517383884,56.2500000000001,19.3911166878577));
#2997=CARTESIAN_POINT('',(-13.9167517383884,56.25,10.3911166878578));
#2998=CARTESIAN_POINT('',(-6.41675173838841,56.2500000000001,19.3911166878577));
#2999=CARTESIAN_POINT('',(-13.9167517383884,56.2500000000001,19.3911166878577));
#3000=CARTESIAN_POINT('',(-6.41675173838841,56.2500000000001,19.3911166878577));
#3001=CARTESIAN_POINT('',(23.5832482616121,56.2500000000001,19.3911166878577));
#3002=CARTESIAN_POINT('',(23.5832482616121,56.2500000000001,19.3911166878577));
#3003=CARTESIAN_POINT('',(43.0832482616116,56.2500000000001,19.3911166878577));
#3004=CARTESIAN_POINT('',(-13.9167517383884,56.2500000000001,19.3911166878577));
#3005=CARTESIAN_POINT('',(43.0832482616116,56.2500000000001,19.3911166878577));
#3006=CARTESIAN_POINT('',(61.0832482616116,56.2500000000001,19.3911166878577));
#3007=CARTESIAN_POINT('',(61.0832482616116,56.2500000000001,19.3911166878577));
#3008=CARTESIAN_POINT('',(-13.9167517383884,56.2500000000001,19.3911166878577));
#3009=CARTESIAN_POINT('Origin',(-13.9167517383884,56.25,10.3911166878578));
#3010=CARTESIAN_POINT('',(-13.9167517383884,-11.25,19.3911166878577));
#3011=CARTESIAN_POINT('',(-13.9167517383884,-11.25,10.3911166878578));
#3012=CARTESIAN_POINT('',(-13.9167517383884,-11.25,19.3911166878577));
#3013=CARTESIAN_POINT('Origin',(-13.9167517383884,-11.25,10.3911166878578));
#3014=CARTESIAN_POINT('',(61.0832482616116,-11.25,19.3911166878577));
#3015=CARTESIAN_POINT('',(-13.9167517383884,-11.25,19.3911166878577));
#3016=CARTESIAN_POINT('',(61.0832482616116,-11.25,19.3911166878577));
#3017=CARTESIAN_POINT('',(43.0832482616116,-11.25,19.3911166878577));
#3018=CARTESIAN_POINT('',(43.0832482616116,-11.25,19.3911166878577));
#3019=CARTESIAN_POINT('',(23.5832482616121,-11.25,19.3911166878578));
#3020=CARTESIAN_POINT('',(-13.9167517383884,-11.25,19.3911166878577));
#3021=CARTESIAN_POINT('',(23.5832482616121,-11.25,19.3911166878578));
#3022=CARTESIAN_POINT('',(-6.41675173838841,-11.25,19.3911166878578));
#3023=CARTESIAN_POINT('',(-6.41675173838841,-11.25,19.3911166878578));
#3024=CARTESIAN_POINT('',(-13.9167517383884,-11.25,19.3911166878577));
#3025=CARTESIAN_POINT('Origin',(23.5832482616121,-11.25,19.3911166878578));
#3026=CARTESIAN_POINT('',(23.5832482616121,-11.25,19.3911166878578));
#3027=CARTESIAN_POINT('Origin',(43.0832482616116,-11.25,19.3911166878577));
#3028=CARTESIAN_POINT('',(43.0832482616116,-11.25,19.3911166878577));
#3029=CARTESIAN_POINT('Origin',(-13.9167517383884,-11.25,19.3911166878577));
#3030=CARTESIAN_POINT('Origin',(-6.41675173838841,-11.25,19.3911166878578));
#3031=CARTESIAN_POINT('',(-6.41675173838841,-11.25,19.3911166878578));
#3032=CARTESIAN_POINT('Origin',(-13.9167517383884,-11.25,19.3911166878577));
#3033=CARTESIAN_POINT('Origin',(61.0832482616116,-11.25,19.3911166878577));
#3034=CARTESIAN_POINT('',(61.0832482616116,-11.25,19.3911166878577));
#3035=CARTESIAN_POINT('Origin',(-13.9167517383884,-11.25,19.3911166878577));
#3193=UNCERTAINTY_MEASURE_WITH_UNIT(LENGTH_MEASURE(0.01),#3207,
'DISTANCE_ACCURACY_VALUE',
'Maximum model space distance between geometric entities at asserted c
onnectivities');
#3196=UNCERTAINTY_MEASURE_WITH_UNIT(LENGTH_MEASURE(0.01),#3207,
'DISTANCE_ACCURACY_VALUE',
'Maximum model space distance between geometric entities at asserted c
onnectivities');
#3203=(
GEOMETRIC_REPRESENTATION_CONTEXT(3)
GLOBAL_UNCERTAINTY_ASSIGNED_CONTEXT((#3193))
GLOBAL_UNIT_ASSIGNED_CONTEXT((#3207,#3209,#3210))
REPRESENTATION_CONTEXT('','3D')
);
#3206=(
GEOMETRIC_REPRESENTATION_CONTEXT(3)
GLOBAL_UNCERTAINTY_ASSIGNED_CONTEXT((#3196))
GLOBAL_UNIT_ASSIGNED_CONTEXT((#3207,#3209,#3210))
REPRESENTATION_CONTEXT('','3D')
);
#3207=(
LENGTH_UNIT()
NAMED_UNIT(*)
SI_UNIT(.MILLI.,.METRE.)
);
#3209=(
NAMED_UNIT(*)
PLANE_ANGLE_UNIT()
SI_UNIT($,.RADIAN.)
);
#3210=(
NAMED_UNIT(*)
SI_UNIT($,.STERADIAN.)
SOLID_ANGLE_UNIT()
);
#3217=SHAPE_DEFINITION_REPRESENTATION(#3226,#3244);
#3226=PRODUCT_DEFINITION_SHAPE('',$,#3254);
#3244=SHAPE_REPRESENTATION('',(#1983),#3203);
#3247=PRODUCT_DEFINITION_CONTEXT('part definition',#3276,'design');
#3254=PRODUCT_DEFINITION('Base Block','Base Block',#3263,#3247);
#3263=PRODUCT_DEFINITION_FORMATION('',$,#3284);
#3276=APPLICATION_CONTEXT(
'Core Data for Automotive Mechanical Design Process');
#3277=PRODUCT_CONTEXT('part definition',#3276,'mechanical');
#3284=PRODUCT('Base Block','Base Block',$,(#3277));
#3289=PRESENTATION_STYLE_ASSIGNMENT((#3293));
#3293=SURFACE_STYLE_USAGE(.BOTH.,#3297);
#3297=SURFACE_SIDE_STYLE('',(#3301));
#3301=SURFACE_STYLE_FILL_AREA(#3305);
#3305=FILL_AREA_STYLE('Opaque(97,158,199)',(#3309));
#3309=FILL_AREA_STYLE_COLOUR('Opaque(97,158,199)',#3313);
#3313=COLOUR_RGB('Opaque(97,158,199)',0.380392156862745,0.619607843137255,
0.780392156862745);
ENDSEC;
END-ISO-10303-21;
